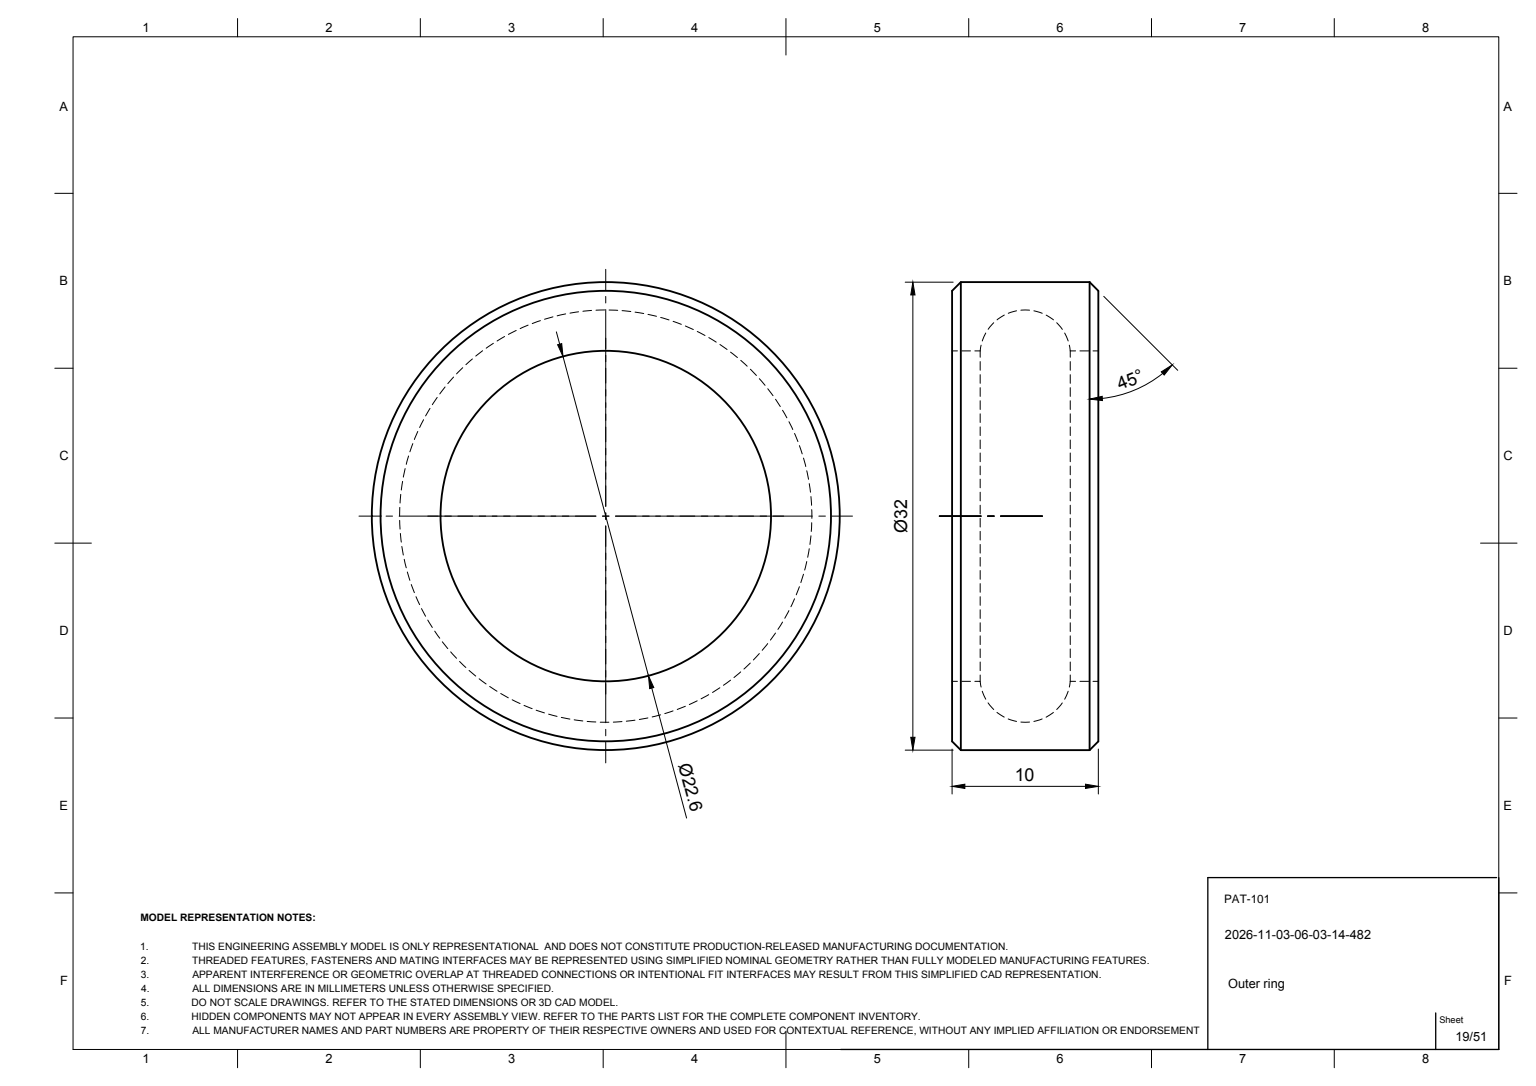
ISO-10303-21;
HEADER;
/* Generated by software containing ST-Developer
 * from STEP Tools, Inc. (www.steptools.com) 
 */

FILE_DESCRIPTION(
/* description */ ('Spur gear reduction stage 2-1 on bearing plates'),
/* implementation_level */ '2;1');

FILE_NAME(
/* name */ 'Outer ring.step',
/* time_stamp */ '2026-10-28T03:22:07-07:00',
/* author */ (''),
/* organization */ (''),
/* preprocessor_version */ 'ST-DEVELOPER v20.2',
/* originating_system */ 'Autodesk Translation Framework v15.17.0.0',
/* authorisation */ '');

FILE_SCHEMA (('AUTOMOTIVE_DESIGN { 1 0 10303 214 3 1 1 }'));
ENDSEC;

DATA;
#10=MECHANICAL_DESIGN_GEOMETRIC_PRESENTATION_REPRESENTATION('',(#961),#53909);
#826=TOROIDAL_SURFACE('',#12175,1.1,0.309556);
#842=CONICAL_SURFACE('',#12186,1.57,0.785398163397449);
#843=CONICAL_SURFACE('',#12190,1.57,0.785398163397449);
#875=SHAPE_REPRESENTATION_RELATIONSHIP('SRR','None',#54103,#918);
#918=ADVANCED_BREP_SHAPE_REPRESENTATION('',(#1017),#53877);
#961=STYLED_ITEM('',(#54397),#1017);
#1017=MANIFOLD_SOLID_BREP('Body1',#11287);
#1180=FACE_BOUND('',#2446,.T.);
#1181=FACE_BOUND('',#2451,.T.);
#1316=PLANE('',#12183);
#1317=PLANE('',#12192);
#1675=FACE_OUTER_BOUND('',#2443,.T.);
#1676=FACE_OUTER_BOUND('',#2444,.T.);
#1677=FACE_OUTER_BOUND('',#2445,.T.);
#1678=FACE_OUTER_BOUND('',#2447,.T.);
#1679=FACE_OUTER_BOUND('',#2448,.T.);
#1680=FACE_OUTER_BOUND('',#2449,.T.);
#1681=FACE_OUTER_BOUND('',#2450,.T.);
#1682=FACE_OUTER_BOUND('',#2452,.T.);
#2443=EDGE_LOOP('',(#8040,#8041,#8042,#8043,#8044,#8045));
#2444=EDGE_LOOP('',(#8046,#8047,#8048,#8049,#8050));
#2445=EDGE_LOOP('',(#8051));
#2446=EDGE_LOOP('',(#8052));
#2447=EDGE_LOOP('',(#8053,#8054,#8055,#8056));
#2448=EDGE_LOOP('',(#8057,#8058,#8059,#8060));
#2449=EDGE_LOOP('',(#8061,#8062,#8063,#8064));
#2450=EDGE_LOOP('',(#8065));
#2451=EDGE_LOOP('',(#8066));
#2452=EDGE_LOOP('',(#8067,#8068,#8069,#8070,#8071));
#3142=LINE('',#16748,#3783);
#3143=LINE('',#16757,#3784);
#3144=LINE('',#16761,#3785);
#3145=LINE('',#16765,#3786);
#3146=LINE('',#16768,#3787);
#3783=VECTOR('',#13901,1.129765);
#3784=VECTOR('',#13912,1.57);
#3785=VECTOR('',#13917,1.6);
#3786=VECTOR('',#13922,1.57);
#3787=VECTOR('',#13927,1.129765);
#4438=CIRCLE('',#12176,1.129765);
#4439=CIRCLE('',#12177,1.129765);
#4440=CIRCLE('',#12178,0.309556);
#4441=CIRCLE('',#12179,1.129765);
#4442=CIRCLE('',#12180,1.129765);
#4443=CIRCLE('',#12182,1.129765);
#4444=CIRCLE('',#12184,1.54);
#4445=CIRCLE('',#12185,1.129765);
#4446=CIRCLE('',#12187,1.6);
#4447=CIRCLE('',#12189,1.6);
#4448=CIRCLE('',#12191,1.54);
#5010=VERTEX_POINT('',#16736);
#5011=VERTEX_POINT('',#16737);
#5012=VERTEX_POINT('',#16740);
#5013=VERTEX_POINT('',#16742);
#5014=VERTEX_POINT('',#16746);
#5015=VERTEX_POINT('',#16750);
#5016=VERTEX_POINT('',#16752);
#5017=VERTEX_POINT('',#16755);
#5018=VERTEX_POINT('',#16759);
#5019=VERTEX_POINT('',#16763);
#6162=EDGE_CURVE('',#5010,#5011,#4438,.T.);
#6163=EDGE_CURVE('',#5011,#5010,#4439,.T.);
#6164=EDGE_CURVE('',#5011,#5012,#4440,.T.);
#6165=EDGE_CURVE('',#5013,#5012,#4441,.T.);
#6166=EDGE_CURVE('',#5012,#5013,#4442,.T.);
#6167=EDGE_CURVE('',#5014,#5014,#4443,.T.);
#6168=EDGE_CURVE('',#5014,#5013,#3142,.T.);
#6169=EDGE_CURVE('',#5015,#5015,#4444,.T.);
#6170=EDGE_CURVE('',#5016,#5016,#4445,.T.);
#6171=EDGE_CURVE('',#5017,#5017,#4446,.T.);
#6172=EDGE_CURVE('',#5017,#5015,#3143,.T.);
#6173=EDGE_CURVE('',#5018,#5018,#4447,.T.);
#6174=EDGE_CURVE('',#5018,#5017,#3144,.T.);
#6175=EDGE_CURVE('',#5019,#5019,#4448,.T.);
#6176=EDGE_CURVE('',#5019,#5018,#3145,.T.);
#6177=EDGE_CURVE('',#5010,#5016,#3146,.T.);
#8040=ORIENTED_EDGE('',*,*,#6162,.F.);
#8041=ORIENTED_EDGE('',*,*,#6163,.F.);
#8042=ORIENTED_EDGE('',*,*,#6164,.T.);
#8043=ORIENTED_EDGE('',*,*,#6165,.F.);
#8044=ORIENTED_EDGE('',*,*,#6166,.F.);
#8045=ORIENTED_EDGE('',*,*,#6164,.F.);
#8046=ORIENTED_EDGE('',*,*,#6167,.T.);
#8047=ORIENTED_EDGE('',*,*,#6168,.T.);
#8048=ORIENTED_EDGE('',*,*,#6165,.T.);
#8049=ORIENTED_EDGE('',*,*,#6166,.T.);
#8050=ORIENTED_EDGE('',*,*,#6168,.F.);
#8051=ORIENTED_EDGE('',*,*,#6169,.F.);
#8052=ORIENTED_EDGE('',*,*,#6170,.T.);
#8053=ORIENTED_EDGE('',*,*,#6171,.F.);
#8054=ORIENTED_EDGE('',*,*,#6172,.T.);
#8055=ORIENTED_EDGE('',*,*,#6169,.T.);
#8056=ORIENTED_EDGE('',*,*,#6172,.F.);
#8057=ORIENTED_EDGE('',*,*,#6173,.F.);
#8058=ORIENTED_EDGE('',*,*,#6174,.T.);
#8059=ORIENTED_EDGE('',*,*,#6171,.T.);
#8060=ORIENTED_EDGE('',*,*,#6174,.F.);
#8061=ORIENTED_EDGE('',*,*,#6175,.F.);
#8062=ORIENTED_EDGE('',*,*,#6176,.T.);
#8063=ORIENTED_EDGE('',*,*,#6173,.T.);
#8064=ORIENTED_EDGE('',*,*,#6176,.F.);
#8065=ORIENTED_EDGE('',*,*,#6175,.T.);
#8066=ORIENTED_EDGE('',*,*,#6167,.F.);
#8067=ORIENTED_EDGE('',*,*,#6162,.T.);
#8068=ORIENTED_EDGE('',*,*,#6163,.T.);
#8069=ORIENTED_EDGE('',*,*,#6177,.T.);
#8070=ORIENTED_EDGE('',*,*,#6170,.F.);
#8071=ORIENTED_EDGE('',*,*,#6177,.F.);
#10503=CYLINDRICAL_SURFACE('',#12181,1.129765);
#10504=CYLINDRICAL_SURFACE('',#12188,1.6);
#10505=CYLINDRICAL_SURFACE('',#12193,1.129765);
#10795=ADVANCED_FACE('',(#1675),#826,.F.);
#10796=ADVANCED_FACE('',(#1676),#10503,.F.);
#10797=ADVANCED_FACE('',(#1677,#1180),#1316,.T.);
#10798=ADVANCED_FACE('',(#1678),#842,.T.);
#10799=ADVANCED_FACE('',(#1679),#10504,.T.);
#10800=ADVANCED_FACE('',(#1680),#843,.T.);
#10801=ADVANCED_FACE('',(#1681,#1181),#1317,.T.);
#10802=ADVANCED_FACE('',(#1682),#10505,.F.);
#11287=CLOSED_SHELL('',(#10795,#10796,#10797,#10798,#10799,#10800,#10801,
#10802));
#12174=AXIS2_PLACEMENT_3D('',#16734,#13883,#13884);
#12175=AXIS2_PLACEMENT_3D('',#16735,#13885,#13886);
#12176=AXIS2_PLACEMENT_3D('',#16738,#13887,#13888);
#12177=AXIS2_PLACEMENT_3D('',#16739,#13889,#13890);
#12178=AXIS2_PLACEMENT_3D('',#16741,#13891,#13892);
#12179=AXIS2_PLACEMENT_3D('',#16743,#13893,#13894);
#12180=AXIS2_PLACEMENT_3D('',#16744,#13895,#13896);
#12181=AXIS2_PLACEMENT_3D('',#16745,#13897,#13898);
#12182=AXIS2_PLACEMENT_3D('',#16747,#13899,#13900);
#12183=AXIS2_PLACEMENT_3D('',#16749,#13902,#13903);
#12184=AXIS2_PLACEMENT_3D('',#16751,#13904,#13905);
#12185=AXIS2_PLACEMENT_3D('',#16753,#13906,#13907);
#12186=AXIS2_PLACEMENT_3D('',#16754,#13908,#13909);
#12187=AXIS2_PLACEMENT_3D('',#16756,#13910,#13911);
#12188=AXIS2_PLACEMENT_3D('',#16758,#13913,#13914);
#12189=AXIS2_PLACEMENT_3D('',#16760,#13915,#13916);
#12190=AXIS2_PLACEMENT_3D('',#16762,#13918,#13919);
#12191=AXIS2_PLACEMENT_3D('',#16764,#13920,#13921);
#12192=AXIS2_PLACEMENT_3D('',#16766,#13923,#13924);
#12193=AXIS2_PLACEMENT_3D('',#16767,#13925,#13926);
#13883=DIRECTION('axis',(0.,0.,1.));
#13884=DIRECTION('refdir',(1.,0.,0.));
#13885=DIRECTION('center_axis',(0.,-1.,0.));
#13886=DIRECTION('ref_axis',(0.,0.,-1.));
#13887=DIRECTION('center_axis',(0.,-1.,0.));
#13888=DIRECTION('ref_axis',(1.,0.,0.));
#13889=DIRECTION('center_axis',(0.,-1.,0.));
#13890=DIRECTION('ref_axis',(1.,0.,0.));
#13891=DIRECTION('center_axis',(1.,0.,1.22464679914735E-16));
#13892=DIRECTION('ref_axis',(-1.22464679914735E-16,0.,1.));
#13893=DIRECTION('center_axis',(0.,1.,0.));
#13894=DIRECTION('ref_axis',(1.,0.,0.));
#13895=DIRECTION('center_axis',(0.,1.,0.));
#13896=DIRECTION('ref_axis',(1.,0.,0.));
#13897=DIRECTION('center_axis',(0.,-1.,0.));
#13898=DIRECTION('ref_axis',(1.,0.,0.));
#13899=DIRECTION('center_axis',(0.,-1.,0.));
#13900=DIRECTION('ref_axis',(1.,0.,0.));
#13901=DIRECTION('',(0.,1.,0.));
#13902=DIRECTION('center_axis',(0.,1.,0.));
#13903=DIRECTION('ref_axis',(0.,0.,1.));
#13904=DIRECTION('center_axis',(0.,-1.,0.));
#13905=DIRECTION('ref_axis',(1.,0.,0.));
#13906=DIRECTION('center_axis',(0.,-1.,0.));
#13907=DIRECTION('ref_axis',(1.,0.,0.));
#13908=DIRECTION('center_axis',(0.,-1.,0.));
#13909=DIRECTION('ref_axis',(1.,0.,0.));
#13910=DIRECTION('center_axis',(0.,-1.,0.));
#13911=DIRECTION('ref_axis',(1.,0.,0.));
#13912=DIRECTION('',(0.707106781186548,0.707106781186547,8.65956056235494E-17));
#13913=DIRECTION('center_axis',(0.,-1.,0.));
#13914=DIRECTION('ref_axis',(1.,0.,0.));
#13915=DIRECTION('center_axis',(0.,-1.,0.));
#13916=DIRECTION('ref_axis',(1.,0.,0.));
#13917=DIRECTION('',(0.,1.,0.));
#13918=DIRECTION('center_axis',(0.,1.,0.));
#13919=DIRECTION('ref_axis',(1.,0.,0.));
#13920=DIRECTION('center_axis',(0.,-1.,0.));
#13921=DIRECTION('ref_axis',(1.,0.,0.));
#13922=DIRECTION('',(-0.707106781186548,0.707106781186547,-8.65956056235494E-17));
#13923=DIRECTION('center_axis',(0.,-1.,0.));
#13924=DIRECTION('ref_axis',(0.,0.,-1.));
#13925=DIRECTION('center_axis',(0.,-1.,0.));
#13926=DIRECTION('ref_axis',(1.,0.,0.));
#13927=DIRECTION('',(0.,1.,0.));
#16734=CARTESIAN_POINT('',(0.,0.,0.));
#16735=CARTESIAN_POINT('Origin',(0.,0.,0.));
#16736=CARTESIAN_POINT('',(-1.129765,0.308121667383195,-1.38356309103871E-16));
#16737=CARTESIAN_POINT('',(-1.38356309103871E-16,0.308121667383195,1.129765));
#16738=CARTESIAN_POINT('Origin',(0.,0.308121667383195,0.));
#16739=CARTESIAN_POINT('Origin',(0.,0.308121667383195,0.));
#16740=CARTESIAN_POINT('',(-1.38356309103871E-16,-0.308121667383195,1.129765));
#16741=CARTESIAN_POINT('Origin',(-1.34711147906209E-16,0.,1.1));
#16742=CARTESIAN_POINT('',(-1.129765,-0.308121667383195,1.38356309103871E-16));
#16743=CARTESIAN_POINT('Origin',(0.,-0.308121667383195,0.));
#16744=CARTESIAN_POINT('Origin',(0.,-0.308121667383195,0.));
#16745=CARTESIAN_POINT('Origin',(0.,0.,0.));
#16746=CARTESIAN_POINT('',(-1.129765,-0.5,-1.38356309103871E-16));
#16747=CARTESIAN_POINT('Origin',(0.,-0.5,0.));
#16748=CARTESIAN_POINT('',(-1.129765,0.,-1.38356309103871E-16));
#16749=CARTESIAN_POINT('Origin',(1.54,0.5,0.));
#16750=CARTESIAN_POINT('',(-1.54,0.5,-1.88595607068692E-16));
#16751=CARTESIAN_POINT('Origin',(0.,0.5,0.));
#16752=CARTESIAN_POINT('',(-1.129765,0.5,-1.38356309103871E-16));
#16753=CARTESIAN_POINT('Origin',(0.,0.5,0.));
#16754=CARTESIAN_POINT('Origin',(0.,0.47,0.));
#16755=CARTESIAN_POINT('',(-1.6,0.44,-1.95943487863577E-16));
#16756=CARTESIAN_POINT('Origin',(0.,0.44,0.));
#16757=CARTESIAN_POINT('',(-1.57,0.47,-1.92269547466134E-16));
#16758=CARTESIAN_POINT('Origin',(0.,0.,0.));
#16759=CARTESIAN_POINT('',(-1.6,-0.44,-1.95943487863577E-16));
#16760=CARTESIAN_POINT('Origin',(0.,-0.44,0.));
#16761=CARTESIAN_POINT('',(-1.6,0.,-1.95943487863577E-16));
#16762=CARTESIAN_POINT('Origin',(0.,-0.47,0.));
#16763=CARTESIAN_POINT('',(-1.54,-0.5,-1.88595607068692E-16));
#16764=CARTESIAN_POINT('Origin',(0.,-0.5,0.));
#16765=CARTESIAN_POINT('',(-1.57,-0.47,-1.92269547466134E-16));
#16766=CARTESIAN_POINT('Origin',(1.129765,-0.5,0.));
#16767=CARTESIAN_POINT('Origin',(0.,0.,0.));
#16768=CARTESIAN_POINT('',(-1.129765,0.,-1.38356309103871E-16));
#53827=UNCERTAINTY_MEASURE_WITH_UNIT(LENGTH_MEASURE(0.001),#53910,
'DISTANCE_ACCURACY_VALUE',
'Maximum model space distance between geometric entities at asserted c
onnectivities');
#53859=UNCERTAINTY_MEASURE_WITH_UNIT(LENGTH_MEASURE(0.001),#53910,
'DISTANCE_ACCURACY_VALUE',
'Maximum model space distance between geometric entities at asserted c
onnectivities');
#53877=(
GEOMETRIC_REPRESENTATION_CONTEXT(3)
GLOBAL_UNCERTAINTY_ASSIGNED_CONTEXT((#53827))
GLOBAL_UNIT_ASSIGNED_CONTEXT((#53910,#53912,#53913))
REPRESENTATION_CONTEXT('','3D')
);
#53909=(
GEOMETRIC_REPRESENTATION_CONTEXT(3)
GLOBAL_UNCERTAINTY_ASSIGNED_CONTEXT((#53859))
GLOBAL_UNIT_ASSIGNED_CONTEXT((#53910,#53912,#53913))
REPRESENTATION_CONTEXT('','3D')
);
#53910=(
LENGTH_UNIT()
NAMED_UNIT(*)
SI_UNIT(.CENTI.,.METRE.)
);
#53912=(
NAMED_UNIT(*)
PLANE_ANGLE_UNIT()
SI_UNIT($,.RADIAN.)
);
#53913=(
NAMED_UNIT(*)
SI_UNIT($,.STERADIAN.)
SOLID_ANGLE_UNIT()
);
#53931=SHAPE_DEFINITION_REPRESENTATION(#53980,#54103);
#53980=PRODUCT_DEFINITION_SHAPE('',$,#54153);
#54103=SHAPE_REPRESENTATION('',(#12174),#53877);
#54135=PRODUCT_DEFINITION_CONTEXT('part definition',#54284,'design');
#54153=PRODUCT_DEFINITION('Outer ring','Outer ring',#54202,#54135);
#54202=PRODUCT_DEFINITION_FORMATION('',$,#54303);
#54284=APPLICATION_CONTEXT(
'Core Data for Automotive Mechanical Design Process');
#54285=PRODUCT_CONTEXT('part definition',#54284,'mechanical');
#54303=PRODUCT('Outer ring','Outer ring','Outer ring',(#54285));
#54391=COLOUR_RGB('Grey',0.48,0.52,0.57);
#54392=FILL_AREA_STYLE_COLOUR('',#54391);
#54393=FILL_AREA_STYLE('',(#54392));
#54394=SURFACE_STYLE_FILL_AREA(#54393);
#54395=SURFACE_SIDE_STYLE('',(#54394));
#54396=SURFACE_STYLE_USAGE(.BOTH.,#54395);
#54397=PRESENTATION_STYLE_ASSIGNMENT((#54396));
ENDSEC;
END-ISO-10303-21;
